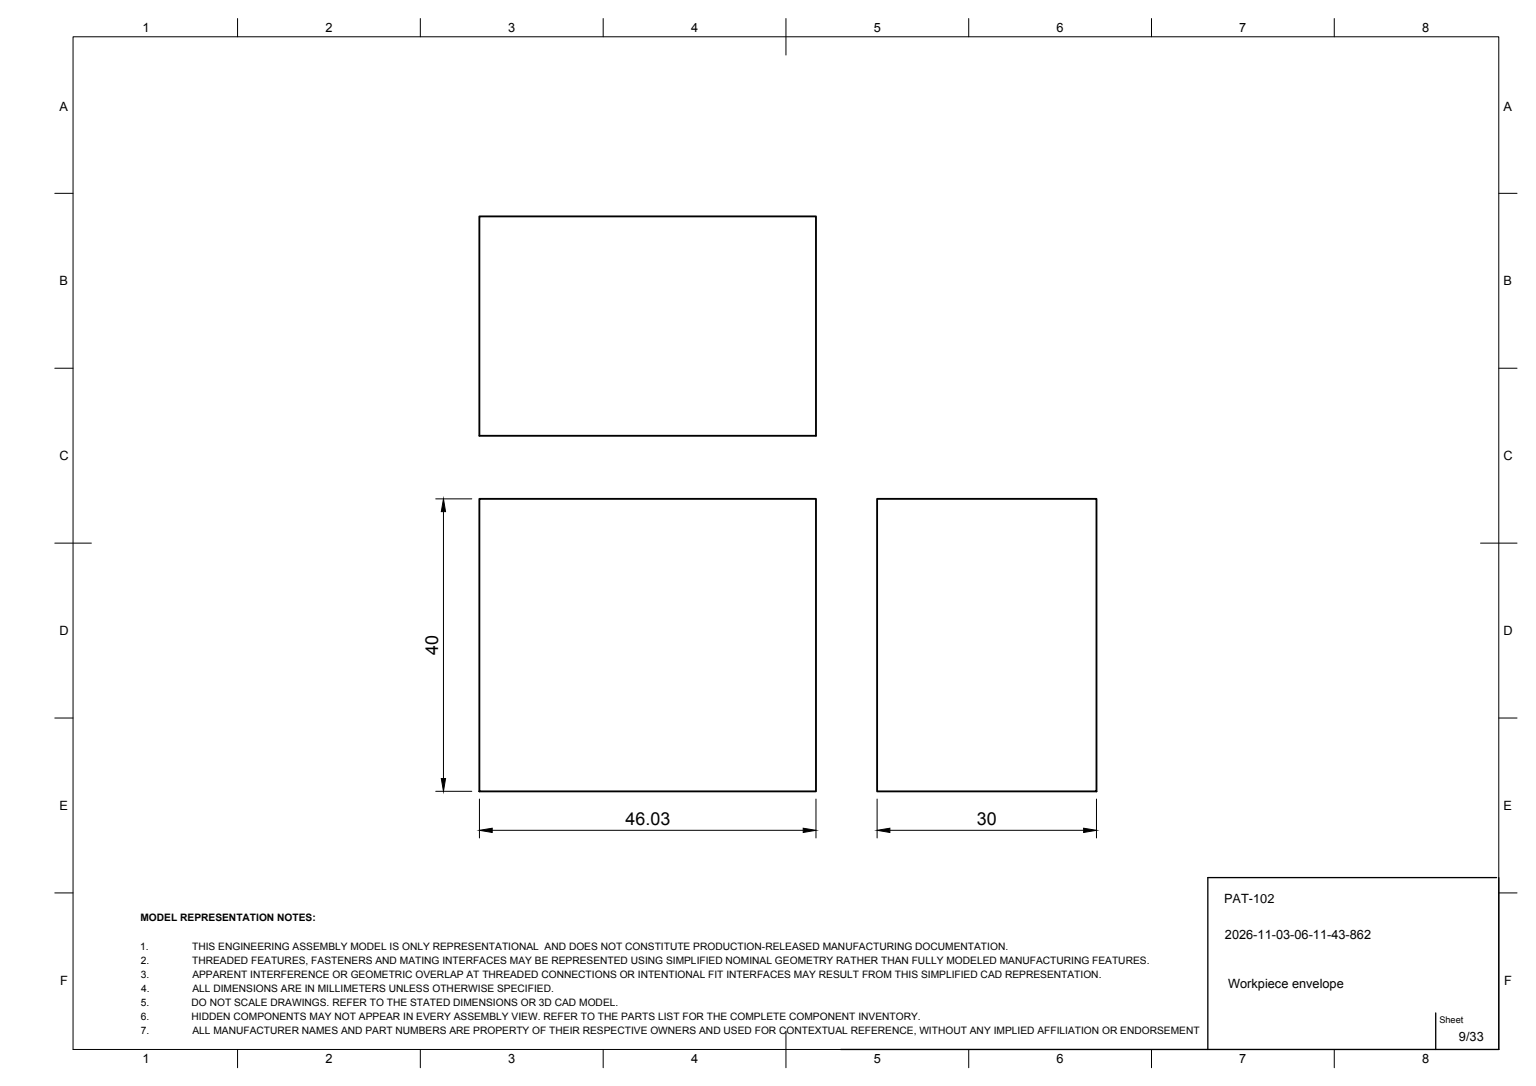
ISO-10303-21;
HEADER;
/* Generated by software containing ST-Developer
 * from STEP Tools, Inc. (www.steptools.com) 
 */

FILE_DESCRIPTION(
/* description */ ('Swing-away clamp arm'),
/* implementation_level */ '2;1');

FILE_NAME(
/* name */ 'Workpiece envelope.step',
/* time_stamp */ '2026-10-28T03:26:03-07:00',
/* author */ (''),
/* organization */ (''),
/* preprocessor_version */ 'ST-DEVELOPER v20.2',
/* originating_system */ 'Autodesk Translation Framework v15.17.0.0',
/* authorisation */ '');

FILE_SCHEMA (('AUTOMOTIVE_DESIGN { 1 0 10303 214 3 1 1 }'));
ENDSEC;

DATA;
#10=MECHANICAL_DESIGN_GEOMETRIC_PRESENTATION_REPRESENTATION('',(#297),#10627);
#245=SHAPE_REPRESENTATION_RELATIONSHIP('SRR','None',#10743,#271);
#271=ADVANCED_BREP_SHAPE_REPRESENTATION('',(#331),#10602);
#297=STYLED_ITEM('',(#10958),#331);
#331=MANIFOLD_SOLID_BREP('Body1',#4903);
#518=PLANE('',#5360);
#519=PLANE('',#5361);
#520=PLANE('',#5362);
#521=PLANE('',#5363);
#522=PLANE('',#5364);
#523=PLANE('',#5365);
#716=FACE_OUTER_BOUND('',#1049,.T.);
#717=FACE_OUTER_BOUND('',#1050,.T.);
#718=FACE_OUTER_BOUND('',#1051,.T.);
#719=FACE_OUTER_BOUND('',#1052,.T.);
#720=FACE_OUTER_BOUND('',#1053,.T.);
#721=FACE_OUTER_BOUND('',#1054,.T.);
#1049=EDGE_LOOP('',(#3669,#3670,#3671,#3672));
#1050=EDGE_LOOP('',(#3673,#3674,#3675,#3676));
#1051=EDGE_LOOP('',(#3677,#3678,#3679,#3680));
#1052=EDGE_LOOP('',(#3681,#3682,#3683,#3684));
#1053=EDGE_LOOP('',(#3685,#3686,#3687,#3688));
#1054=EDGE_LOOP('',(#3689,#3690,#3691,#3692));
#1494=LINE('',#7898,#1816);
#1495=LINE('',#7900,#1817);
#1496=LINE('',#7902,#1818);
#1497=LINE('',#7903,#1819);
#1498=LINE('',#7906,#1820);
#1499=LINE('',#7908,#1821);
#1500=LINE('',#7909,#1822);
#1501=LINE('',#7912,#1823);
#1502=LINE('',#7914,#1824);
#1503=LINE('',#7915,#1825);
#1504=LINE('',#7917,#1826);
#1505=LINE('',#7918,#1827);
#1816=VECTOR('',#6289,1.);
#1817=VECTOR('',#6290,1.);
#1818=VECTOR('',#6291,1.);
#1819=VECTOR('',#6292,1.);
#1820=VECTOR('',#6295,1.);
#1821=VECTOR('',#6296,1.);
#1822=VECTOR('',#6297,1.);
#1823=VECTOR('',#6300,1.);
#1824=VECTOR('',#6301,1.);
#1825=VECTOR('',#6302,1.);
#1826=VECTOR('',#6305,1.);
#1827=VECTOR('',#6306,1.);
#2391=VERTEX_POINT('',#7896);
#2392=VERTEX_POINT('',#7897);
#2393=VERTEX_POINT('',#7899);
#2394=VERTEX_POINT('',#7901);
#2395=VERTEX_POINT('',#7905);
#2396=VERTEX_POINT('',#7907);
#2397=VERTEX_POINT('',#7911);
#2398=VERTEX_POINT('',#7913);
#2867=EDGE_CURVE('',#2391,#2392,#1494,.T.);
#2868=EDGE_CURVE('',#2392,#2393,#1495,.T.);
#2869=EDGE_CURVE('',#2394,#2393,#1496,.T.);
#2870=EDGE_CURVE('',#2391,#2394,#1497,.T.);
#2871=EDGE_CURVE('',#2395,#2391,#1498,.T.);
#2872=EDGE_CURVE('',#2396,#2394,#1499,.T.);
#2873=EDGE_CURVE('',#2395,#2396,#1500,.T.);
#2874=EDGE_CURVE('',#2397,#2395,#1501,.T.);
#2875=EDGE_CURVE('',#2398,#2396,#1502,.T.);
#2876=EDGE_CURVE('',#2397,#2398,#1503,.T.);
#2877=EDGE_CURVE('',#2392,#2397,#1504,.T.);
#2878=EDGE_CURVE('',#2393,#2398,#1505,.T.);
#3669=ORIENTED_EDGE('',*,*,#2867,.T.);
#3670=ORIENTED_EDGE('',*,*,#2868,.T.);
#3671=ORIENTED_EDGE('',*,*,#2869,.F.);
#3672=ORIENTED_EDGE('',*,*,#2870,.F.);
#3673=ORIENTED_EDGE('',*,*,#2871,.T.);
#3674=ORIENTED_EDGE('',*,*,#2870,.T.);
#3675=ORIENTED_EDGE('',*,*,#2872,.F.);
#3676=ORIENTED_EDGE('',*,*,#2873,.F.);
#3677=ORIENTED_EDGE('',*,*,#2874,.T.);
#3678=ORIENTED_EDGE('',*,*,#2873,.T.);
#3679=ORIENTED_EDGE('',*,*,#2875,.F.);
#3680=ORIENTED_EDGE('',*,*,#2876,.F.);
#3681=ORIENTED_EDGE('',*,*,#2877,.T.);
#3682=ORIENTED_EDGE('',*,*,#2876,.T.);
#3683=ORIENTED_EDGE('',*,*,#2878,.F.);
#3684=ORIENTED_EDGE('',*,*,#2868,.F.);
#3685=ORIENTED_EDGE('',*,*,#2878,.T.);
#3686=ORIENTED_EDGE('',*,*,#2875,.T.);
#3687=ORIENTED_EDGE('',*,*,#2872,.T.);
#3688=ORIENTED_EDGE('',*,*,#2869,.T.);
#3689=ORIENTED_EDGE('',*,*,#2877,.F.);
#3690=ORIENTED_EDGE('',*,*,#2867,.F.);
#3691=ORIENTED_EDGE('',*,*,#2871,.F.);
#3692=ORIENTED_EDGE('',*,*,#2874,.F.);
#4671=ADVANCED_FACE('',(#716),#518,.T.);
#4672=ADVANCED_FACE('',(#717),#519,.T.);
#4673=ADVANCED_FACE('',(#718),#520,.T.);
#4674=ADVANCED_FACE('',(#719),#521,.T.);
#4675=ADVANCED_FACE('',(#720),#522,.T.);
#4676=ADVANCED_FACE('',(#721),#523,.F.);
#4903=CLOSED_SHELL('',(#4671,#4672,#4673,#4674,#4675,#4676));
#5359=AXIS2_PLACEMENT_3D('',#7894,#6285,#6286);
#5360=AXIS2_PLACEMENT_3D('',#7895,#6287,#6288);
#5361=AXIS2_PLACEMENT_3D('',#7904,#6293,#6294);
#5362=AXIS2_PLACEMENT_3D('',#7910,#6298,#6299);
#5363=AXIS2_PLACEMENT_3D('',#7916,#6303,#6304);
#5364=AXIS2_PLACEMENT_3D('',#7919,#6307,#6308);
#5365=AXIS2_PLACEMENT_3D('',#7920,#6309,#6310);
#6285=DIRECTION('axis',(0.,0.,1.));
#6286=DIRECTION('refdir',(1.,0.,0.));
#6287=DIRECTION('center_axis',(0.,1.,0.));
#6288=DIRECTION('ref_axis',(-1.,0.,0.));
#6289=DIRECTION('',(-1.,0.,0.));
#6290=DIRECTION('',(0.,0.,1.));
#6291=DIRECTION('',(-1.,0.,0.));
#6292=DIRECTION('',(0.,0.,1.));
#6293=DIRECTION('center_axis',(1.,0.,0.));
#6294=DIRECTION('ref_axis',(0.,1.,0.));
#6295=DIRECTION('',(0.,1.,0.));
#6296=DIRECTION('',(0.,1.,0.));
#6297=DIRECTION('',(0.,0.,1.));
#6298=DIRECTION('center_axis',(0.,-1.,0.));
#6299=DIRECTION('ref_axis',(1.,0.,0.));
#6300=DIRECTION('',(1.,0.,0.));
#6301=DIRECTION('',(1.,0.,0.));
#6302=DIRECTION('',(0.,0.,1.));
#6303=DIRECTION('center_axis',(-1.,0.,0.));
#6304=DIRECTION('ref_axis',(0.,-1.,0.));
#6305=DIRECTION('',(0.,-1.,0.));
#6306=DIRECTION('',(0.,-1.,0.));
#6307=DIRECTION('center_axis',(0.,0.,1.));
#6308=DIRECTION('ref_axis',(1.,0.,0.));
#6309=DIRECTION('center_axis',(0.,0.,1.));
#6310=DIRECTION('ref_axis',(1.,0.,0.));
#7894=CARTESIAN_POINT('',(0.,0.,0.));
#7895=CARTESIAN_POINT('Origin',(14.,1.5,1.));
#7896=CARTESIAN_POINT('',(14.,1.5,1.));
#7897=CARTESIAN_POINT('',(10.,1.5,1.));
#7898=CARTESIAN_POINT('',(14.,1.5,1.));
#7899=CARTESIAN_POINT('',(10.,1.5,5.60303845));
#7900=CARTESIAN_POINT('',(10.,1.5,1.));
#7901=CARTESIAN_POINT('',(14.,1.5,5.60303845));
#7902=CARTESIAN_POINT('',(14.,1.5,5.60303845));
#7903=CARTESIAN_POINT('',(14.,1.5,1.));
#7904=CARTESIAN_POINT('Origin',(14.,-1.5,1.));
#7905=CARTESIAN_POINT('',(14.,-1.5,1.));
#7906=CARTESIAN_POINT('',(14.,-1.5,1.));
#7907=CARTESIAN_POINT('',(14.,-1.5,5.60303845));
#7908=CARTESIAN_POINT('',(14.,-1.5,5.60303845));
#7909=CARTESIAN_POINT('',(14.,-1.5,1.));
#7910=CARTESIAN_POINT('Origin',(10.,-1.5,1.));
#7911=CARTESIAN_POINT('',(10.,-1.5,1.));
#7912=CARTESIAN_POINT('',(10.,-1.5,1.));
#7913=CARTESIAN_POINT('',(10.,-1.5,5.60303845));
#7914=CARTESIAN_POINT('',(10.,-1.5,5.60303845));
#7915=CARTESIAN_POINT('',(10.,-1.5,1.));
#7916=CARTESIAN_POINT('Origin',(10.,1.5,1.));
#7917=CARTESIAN_POINT('',(10.,1.5,1.));
#7918=CARTESIAN_POINT('',(10.,1.5,5.60303845));
#7919=CARTESIAN_POINT('Origin',(12.,0.,5.60303845));
#7920=CARTESIAN_POINT('Origin',(12.,0.,1.));
#10570=UNCERTAINTY_MEASURE_WITH_UNIT(LENGTH_MEASURE(0.001),#10628,
'DISTANCE_ACCURACY_VALUE',
'Maximum model space distance between geometric entities at asserted c
onnectivities');
#10595=UNCERTAINTY_MEASURE_WITH_UNIT(LENGTH_MEASURE(0.001),#10628,
'DISTANCE_ACCURACY_VALUE',
'Maximum model space distance between geometric entities at asserted c
onnectivities');
#10602=(
GEOMETRIC_REPRESENTATION_CONTEXT(3)
GLOBAL_UNCERTAINTY_ASSIGNED_CONTEXT((#10570))
GLOBAL_UNIT_ASSIGNED_CONTEXT((#10628,#10630,#10631))
REPRESENTATION_CONTEXT('','3D')
);
#10627=(
GEOMETRIC_REPRESENTATION_CONTEXT(3)
GLOBAL_UNCERTAINTY_ASSIGNED_CONTEXT((#10595))
GLOBAL_UNIT_ASSIGNED_CONTEXT((#10628,#10630,#10631))
REPRESENTATION_CONTEXT('','3D')
);
#10628=(
LENGTH_UNIT()
NAMED_UNIT(*)
SI_UNIT(.CENTI.,.METRE.)
);
#10630=(
NAMED_UNIT(*)
PLANE_ANGLE_UNIT()
SI_UNIT($,.RADIAN.)
);
#10631=(
NAMED_UNIT(*)
SI_UNIT($,.STERADIAN.)
SOLID_ANGLE_UNIT()
);
#10638=SHAPE_DEFINITION_REPRESENTATION(#10669,#10743);
#10669=PRODUCT_DEFINITION_SHAPE('',$,#10775);
#10743=SHAPE_REPRESENTATION('',(#5359),#10602);
#10768=PRODUCT_DEFINITION_CONTEXT('part definition',#10863,'design');
#10775=PRODUCT_DEFINITION('Workpiece envelope','Workpiece envelope',#10806,
#10768);
#10806=PRODUCT_DEFINITION_FORMATION('',$,#10871);
#10863=APPLICATION_CONTEXT(
'Core Data for Automotive Mechanical Design Process');
#10864=PRODUCT_CONTEXT('part definition',#10863,'mechanical');
#10871=PRODUCT('Workpiece envelope','Workpiece envelope',
'Workpiece envelope',(#10864));
#10952=COLOUR_RGB('Sky Blue',0.24,0.69,0.87);
#10953=FILL_AREA_STYLE_COLOUR('',#10952);
#10954=FILL_AREA_STYLE('',(#10953));
#10955=SURFACE_STYLE_FILL_AREA(#10954);
#10956=SURFACE_SIDE_STYLE('',(#10955));
#10957=SURFACE_STYLE_USAGE(.BOTH.,#10956);
#10958=PRESENTATION_STYLE_ASSIGNMENT((#10957));
ENDSEC;
END-ISO-10303-21;
